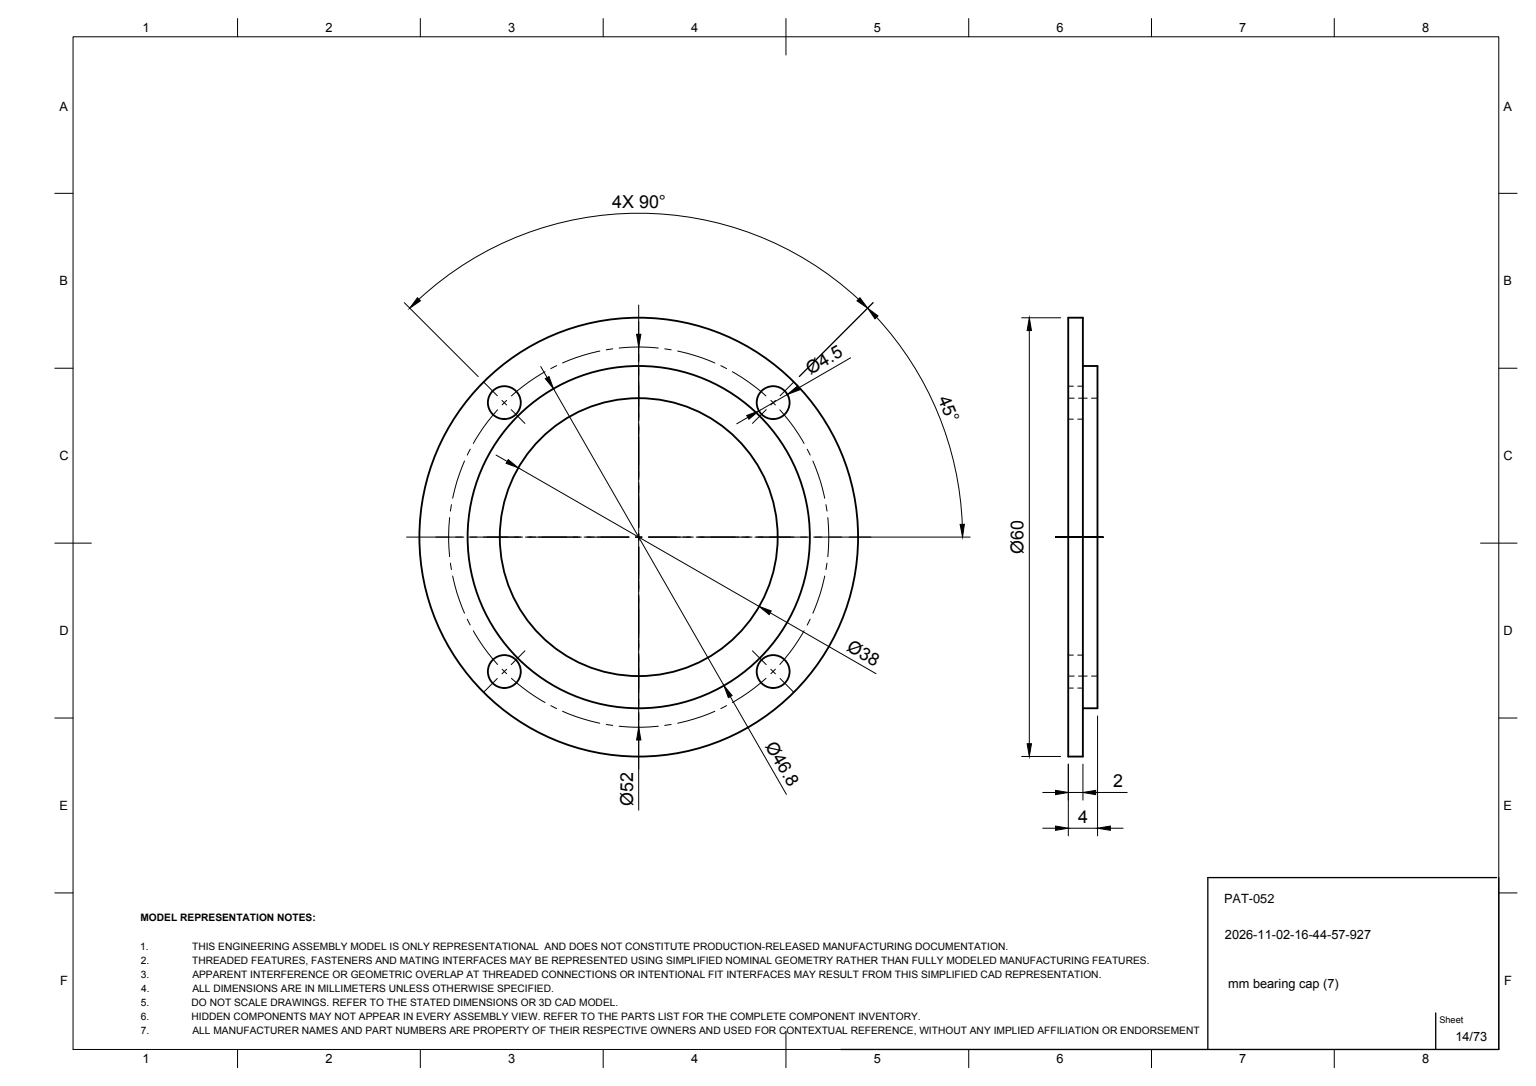
ISO-10303-21;
HEADER;
/* Generated by software containing ST-Developer
 * from STEP Tools, Inc. (www.steptools.com) 
 */

FILE_DESCRIPTION(
/* description */ ('Hand-crank gear train demonstrator'),
/* implementation_level */ '2;1');

FILE_NAME(
/* name */ 'mm bearing cap (7).step',
/* time_stamp */ '2026-10-28T03:22:13-07:00',
/* author */ (''),
/* organization */ (''),
/* preprocessor_version */ 'ST-DEVELOPER v20.2',
/* originating_system */ 'Autodesk Translation Framework v15.17.0.0',
/* authorisation */ '');

FILE_SCHEMA (('AUTOMOTIVE_DESIGN { 1 0 10303 214 3 1 1 }'));
ENDSEC;

DATA;
#10=MECHANICAL_DESIGN_GEOMETRIC_PRESENTATION_REPRESENTATION('',(#1199),#62758);
#1071=SHAPE_REPRESENTATION_RELATIONSHIP('SRR','None',#63043,#1135);
#1135=ADVANCED_BREP_SHAPE_REPRESENTATION('',(#1277),#62697);
#1199=STYLED_ITEM('',(#63462),#1277);
#1277=MANIFOLD_SOLID_BREP('Body1',#16380);
#1476=FACE_BOUND('',#3327,.T.);
#1477=FACE_BOUND('',#3331,.T.);
#1478=FACE_BOUND('',#3332,.T.);
#1479=FACE_BOUND('',#3333,.T.);
#1480=FACE_BOUND('',#3334,.T.);
#1481=FACE_BOUND('',#3335,.T.);
#1482=FACE_BOUND('',#3337,.T.);
#1483=FACE_BOUND('',#3338,.T.);
#1484=FACE_BOUND('',#3339,.T.);
#1485=FACE_BOUND('',#3340,.T.);
#1486=FACE_BOUND('',#3341,.T.);
#1679=PLANE('',#17475);
#1680=PLANE('',#17482);
#1681=PLANE('',#17483);
#2251=FACE_OUTER_BOUND('',#3321,.T.);
#2252=FACE_OUTER_BOUND('',#3322,.T.);
#2253=FACE_OUTER_BOUND('',#3323,.T.);
#2254=FACE_OUTER_BOUND('',#3324,.T.);
#2255=FACE_OUTER_BOUND('',#3325,.T.);
#2256=FACE_OUTER_BOUND('',#3326,.T.);
#2257=FACE_OUTER_BOUND('',#3328,.T.);
#2258=FACE_OUTER_BOUND('',#3329,.T.);
#2259=FACE_OUTER_BOUND('',#3330,.T.);
#2260=FACE_OUTER_BOUND('',#3336,.T.);
#3321=EDGE_LOOP('',(#11417,#11418,#11419,#11420));
#3322=EDGE_LOOP('',(#11421,#11422,#11423,#11424));
#3323=EDGE_LOOP('',(#11425,#11426,#11427,#11428));
#3324=EDGE_LOOP('',(#11429,#11430,#11431,#11432));
#3325=EDGE_LOOP('',(#11433,#11434,#11435,#11436));
#3326=EDGE_LOOP('',(#11437));
#3327=EDGE_LOOP('',(#11438));
#3328=EDGE_LOOP('',(#11439,#11440,#11441,#11442));
#3329=EDGE_LOOP('',(#11443,#11444,#11445,#11446));
#3330=EDGE_LOOP('',(#11447));
#3331=EDGE_LOOP('',(#11448));
#3332=EDGE_LOOP('',(#11449));
#3333=EDGE_LOOP('',(#11450));
#3334=EDGE_LOOP('',(#11451));
#3335=EDGE_LOOP('',(#11452));
#3336=EDGE_LOOP('',(#11453));
#3337=EDGE_LOOP('',(#11454));
#3338=EDGE_LOOP('',(#11455));
#3339=EDGE_LOOP('',(#11456));
#3340=EDGE_LOOP('',(#11457));
#3341=EDGE_LOOP('',(#11458));
#4416=LINE('',#23938,#5548);
#4417=LINE('',#23944,#5549);
#4418=LINE('',#23950,#5550);
#4419=LINE('',#23956,#5551);
#4420=LINE('',#23962,#5552);
#4421=LINE('',#23970,#5553);
#4422=LINE('',#23975,#5554);
#5548=VECTOR('',#19569,0.225000000000001);
#5549=VECTOR('',#19576,0.225000000000001);
#5550=VECTOR('',#19583,0.225000000000001);
#5551=VECTOR('',#19590,0.225000000000001);
#5552=VECTOR('',#19597,2.34);
#5553=VECTOR('',#19608,1.9);
#5554=VECTOR('',#19613,3.);
#6711=CIRCLE('',#17461,0.225000000000001);
#6712=CIRCLE('',#17462,0.225000000000001);
#6713=CIRCLE('',#17464,0.225000000000001);
#6714=CIRCLE('',#17465,0.225000000000001);
#6715=CIRCLE('',#17467,0.225000000000001);
#6716=CIRCLE('',#17468,0.225000000000001);
#6717=CIRCLE('',#17470,0.225000000000001);
#6718=CIRCLE('',#17471,0.225000000000001);
#6719=CIRCLE('',#17473,2.34);
#6720=CIRCLE('',#17474,2.34);
#6721=CIRCLE('',#17476,1.9);
#6722=CIRCLE('',#17478,1.9);
#6723=CIRCLE('',#17480,3.);
#6724=CIRCLE('',#17481,3.);
#7405=VERTEX_POINT('',#23935);
#7406=VERTEX_POINT('',#23937);
#7407=VERTEX_POINT('',#23941);
#7408=VERTEX_POINT('',#23943);
#7409=VERTEX_POINT('',#23947);
#7410=VERTEX_POINT('',#23949);
#7411=VERTEX_POINT('',#23953);
#7412=VERTEX_POINT('',#23955);
#7413=VERTEX_POINT('',#23959);
#7414=VERTEX_POINT('',#23961);
#7415=VERTEX_POINT('',#23965);
#7416=VERTEX_POINT('',#23968);
#7417=VERTEX_POINT('',#23972);
#7418=VERTEX_POINT('',#23974);
#8960=EDGE_CURVE('',#7405,#7405,#6711,.T.);
#8961=EDGE_CURVE('',#7405,#7406,#4416,.T.);
#8962=EDGE_CURVE('',#7406,#7406,#6712,.T.);
#8963=EDGE_CURVE('',#7407,#7407,#6713,.T.);
#8964=EDGE_CURVE('',#7407,#7408,#4417,.T.);
#8965=EDGE_CURVE('',#7408,#7408,#6714,.T.);
#8966=EDGE_CURVE('',#7409,#7409,#6715,.T.);
#8967=EDGE_CURVE('',#7409,#7410,#4418,.T.);
#8968=EDGE_CURVE('',#7410,#7410,#6716,.T.);
#8969=EDGE_CURVE('',#7411,#7411,#6717,.T.);
#8970=EDGE_CURVE('',#7411,#7412,#4419,.T.);
#8971=EDGE_CURVE('',#7412,#7412,#6718,.T.);
#8972=EDGE_CURVE('',#7413,#7413,#6719,.T.);
#8973=EDGE_CURVE('',#7413,#7414,#4420,.T.);
#8974=EDGE_CURVE('',#7414,#7414,#6720,.T.);
#8975=EDGE_CURVE('',#7415,#7415,#6721,.T.);
#8976=EDGE_CURVE('',#7416,#7416,#6722,.T.);
#8977=EDGE_CURVE('',#7416,#7415,#4421,.T.);
#8978=EDGE_CURVE('',#7417,#7417,#6723,.T.);
#8979=EDGE_CURVE('',#7417,#7418,#4422,.T.);
#8980=EDGE_CURVE('',#7418,#7418,#6724,.T.);
#11417=ORIENTED_EDGE('',*,*,#8960,.F.);
#11418=ORIENTED_EDGE('',*,*,#8961,.T.);
#11419=ORIENTED_EDGE('',*,*,#8962,.F.);
#11420=ORIENTED_EDGE('',*,*,#8961,.F.);
#11421=ORIENTED_EDGE('',*,*,#8963,.F.);
#11422=ORIENTED_EDGE('',*,*,#8964,.T.);
#11423=ORIENTED_EDGE('',*,*,#8965,.F.);
#11424=ORIENTED_EDGE('',*,*,#8964,.F.);
#11425=ORIENTED_EDGE('',*,*,#8966,.F.);
#11426=ORIENTED_EDGE('',*,*,#8967,.T.);
#11427=ORIENTED_EDGE('',*,*,#8968,.F.);
#11428=ORIENTED_EDGE('',*,*,#8967,.F.);
#11429=ORIENTED_EDGE('',*,*,#8969,.F.);
#11430=ORIENTED_EDGE('',*,*,#8970,.T.);
#11431=ORIENTED_EDGE('',*,*,#8971,.F.);
#11432=ORIENTED_EDGE('',*,*,#8970,.F.);
#11433=ORIENTED_EDGE('',*,*,#8972,.F.);
#11434=ORIENTED_EDGE('',*,*,#8973,.T.);
#11435=ORIENTED_EDGE('',*,*,#8974,.T.);
#11436=ORIENTED_EDGE('',*,*,#8973,.F.);
#11437=ORIENTED_EDGE('',*,*,#8974,.F.);
#11438=ORIENTED_EDGE('',*,*,#8975,.F.);
#11439=ORIENTED_EDGE('',*,*,#8976,.F.);
#11440=ORIENTED_EDGE('',*,*,#8977,.T.);
#11441=ORIENTED_EDGE('',*,*,#8975,.T.);
#11442=ORIENTED_EDGE('',*,*,#8977,.F.);
#11443=ORIENTED_EDGE('',*,*,#8978,.F.);
#11444=ORIENTED_EDGE('',*,*,#8979,.T.);
#11445=ORIENTED_EDGE('',*,*,#8980,.T.);
#11446=ORIENTED_EDGE('',*,*,#8979,.F.);
#11447=ORIENTED_EDGE('',*,*,#8978,.T.);
#11448=ORIENTED_EDGE('',*,*,#8976,.T.);
#11449=ORIENTED_EDGE('',*,*,#8971,.T.);
#11450=ORIENTED_EDGE('',*,*,#8968,.T.);
#11451=ORIENTED_EDGE('',*,*,#8965,.T.);
#11452=ORIENTED_EDGE('',*,*,#8962,.T.);
#11453=ORIENTED_EDGE('',*,*,#8980,.F.);
#11454=ORIENTED_EDGE('',*,*,#8972,.T.);
#11455=ORIENTED_EDGE('',*,*,#8969,.T.);
#11456=ORIENTED_EDGE('',*,*,#8966,.T.);
#11457=ORIENTED_EDGE('',*,*,#8963,.T.);
#11458=ORIENTED_EDGE('',*,*,#8960,.T.);
#15246=CYLINDRICAL_SURFACE('',#17460,0.225000000000001);
#15247=CYLINDRICAL_SURFACE('',#17463,0.225000000000001);
#15248=CYLINDRICAL_SURFACE('',#17466,0.225000000000001);
#15249=CYLINDRICAL_SURFACE('',#17469,0.225000000000001);
#15250=CYLINDRICAL_SURFACE('',#17472,2.34);
#15251=CYLINDRICAL_SURFACE('',#17477,1.9);
#15252=CYLINDRICAL_SURFACE('',#17479,3.);
#15561=ADVANCED_FACE('',(#2251),#15246,.F.);
#15562=ADVANCED_FACE('',(#2252),#15247,.F.);
#15563=ADVANCED_FACE('',(#2253),#15248,.F.);
#15564=ADVANCED_FACE('',(#2254),#15249,.F.);
#15565=ADVANCED_FACE('',(#2255),#15250,.T.);
#15566=ADVANCED_FACE('',(#2256,#1476),#1679,.F.);
#15567=ADVANCED_FACE('',(#2257),#15251,.F.);
#15568=ADVANCED_FACE('',(#2258),#15252,.T.);
#15569=ADVANCED_FACE('',(#2259,#1477,#1478,#1479,#1480,#1481),#1680,.T.);
#15570=ADVANCED_FACE('',(#2260,#1482,#1483,#1484,#1485,#1486),#1681,.F.);
#16380=CLOSED_SHELL('',(#15561,#15562,#15563,#15564,#15565,#15566,#15567,
#15568,#15569,#15570));
#17459=AXIS2_PLACEMENT_3D('',#23933,#19563,#19564);
#17460=AXIS2_PLACEMENT_3D('',#23934,#19565,#19566);
#17461=AXIS2_PLACEMENT_3D('',#23936,#19567,#19568);
#17462=AXIS2_PLACEMENT_3D('',#23939,#19570,#19571);
#17463=AXIS2_PLACEMENT_3D('',#23940,#19572,#19573);
#17464=AXIS2_PLACEMENT_3D('',#23942,#19574,#19575);
#17465=AXIS2_PLACEMENT_3D('',#23945,#19577,#19578);
#17466=AXIS2_PLACEMENT_3D('',#23946,#19579,#19580);
#17467=AXIS2_PLACEMENT_3D('',#23948,#19581,#19582);
#17468=AXIS2_PLACEMENT_3D('',#23951,#19584,#19585);
#17469=AXIS2_PLACEMENT_3D('',#23952,#19586,#19587);
#17470=AXIS2_PLACEMENT_3D('',#23954,#19588,#19589);
#17471=AXIS2_PLACEMENT_3D('',#23957,#19591,#19592);
#17472=AXIS2_PLACEMENT_3D('',#23958,#19593,#19594);
#17473=AXIS2_PLACEMENT_3D('',#23960,#19595,#19596);
#17474=AXIS2_PLACEMENT_3D('',#23963,#19598,#19599);
#17475=AXIS2_PLACEMENT_3D('',#23964,#19600,#19601);
#17476=AXIS2_PLACEMENT_3D('',#23966,#19602,#19603);
#17477=AXIS2_PLACEMENT_3D('',#23967,#19604,#19605);
#17478=AXIS2_PLACEMENT_3D('',#23969,#19606,#19607);
#17479=AXIS2_PLACEMENT_3D('',#23971,#19609,#19610);
#17480=AXIS2_PLACEMENT_3D('',#23973,#19611,#19612);
#17481=AXIS2_PLACEMENT_3D('',#23976,#19614,#19615);
#17482=AXIS2_PLACEMENT_3D('',#23977,#19616,#19617);
#17483=AXIS2_PLACEMENT_3D('',#23978,#19618,#19619);
#19563=DIRECTION('axis',(0.,0.,1.));
#19564=DIRECTION('refdir',(1.,0.,0.));
#19565=DIRECTION('center_axis',(0.,1.,0.));
#19566=DIRECTION('ref_axis',(1.,0.,0.));
#19567=DIRECTION('center_axis',(0.,1.,0.));
#19568=DIRECTION('ref_axis',(1.,0.,0.));
#19569=DIRECTION('',(0.,1.,0.));
#19570=DIRECTION('center_axis',(0.,-1.,0.));
#19571=DIRECTION('ref_axis',(1.,0.,0.));
#19572=DIRECTION('center_axis',(0.,1.,0.));
#19573=DIRECTION('ref_axis',(1.,0.,0.));
#19574=DIRECTION('center_axis',(0.,1.,0.));
#19575=DIRECTION('ref_axis',(1.,0.,0.));
#19576=DIRECTION('',(0.,1.,0.));
#19577=DIRECTION('center_axis',(0.,-1.,0.));
#19578=DIRECTION('ref_axis',(1.,0.,0.));
#19579=DIRECTION('center_axis',(0.,1.,0.));
#19580=DIRECTION('ref_axis',(1.,0.,0.));
#19581=DIRECTION('center_axis',(0.,1.,0.));
#19582=DIRECTION('ref_axis',(1.,0.,0.));
#19583=DIRECTION('',(0.,1.,0.));
#19584=DIRECTION('center_axis',(0.,-1.,0.));
#19585=DIRECTION('ref_axis',(1.,0.,0.));
#19586=DIRECTION('center_axis',(0.,1.,0.));
#19587=DIRECTION('ref_axis',(1.,0.,0.));
#19588=DIRECTION('center_axis',(0.,1.,0.));
#19589=DIRECTION('ref_axis',(1.,0.,0.));
#19590=DIRECTION('',(0.,1.,0.));
#19591=DIRECTION('center_axis',(0.,-1.,0.));
#19592=DIRECTION('ref_axis',(1.,0.,0.));
#19593=DIRECTION('center_axis',(0.,1.,0.));
#19594=DIRECTION('ref_axis',(1.,0.,0.));
#19595=DIRECTION('center_axis',(0.,1.,0.));
#19596=DIRECTION('ref_axis',(1.,0.,0.));
#19597=DIRECTION('',(0.,-1.,0.));
#19598=DIRECTION('center_axis',(0.,1.,0.));
#19599=DIRECTION('ref_axis',(1.,0.,0.));
#19600=DIRECTION('center_axis',(0.,1.,0.));
#19601=DIRECTION('ref_axis',(1.,0.,0.));
#19602=DIRECTION('center_axis',(0.,-1.,0.));
#19603=DIRECTION('ref_axis',(1.,0.,0.));
#19604=DIRECTION('center_axis',(0.,1.,0.));
#19605=DIRECTION('ref_axis',(1.,0.,0.));
#19606=DIRECTION('center_axis',(0.,-1.,0.));
#19607=DIRECTION('ref_axis',(1.,0.,0.));
#19608=DIRECTION('',(0.,-1.,0.));
#19609=DIRECTION('center_axis',(0.,1.,0.));
#19610=DIRECTION('ref_axis',(1.,0.,0.));
#19611=DIRECTION('center_axis',(0.,1.,0.));
#19612=DIRECTION('ref_axis',(1.,0.,0.));
#19613=DIRECTION('',(0.,-1.,0.));
#19614=DIRECTION('center_axis',(0.,1.,0.));
#19615=DIRECTION('ref_axis',(1.,0.,0.));
#19616=DIRECTION('center_axis',(0.,1.,0.));
#19617=DIRECTION('ref_axis',(1.,0.,0.));
#19618=DIRECTION('center_axis',(0.,1.,0.));
#19619=DIRECTION('ref_axis',(1.,0.,0.));
#23933=CARTESIAN_POINT('',(0.,0.,0.));
#23934=CARTESIAN_POINT('Origin',(16.161522368915,-0.7,7.16152236891498));
#23935=CARTESIAN_POINT('',(15.936522368915,-0.6,7.16152236891498));
#23936=CARTESIAN_POINT('Origin',(16.161522368915,-0.6,7.16152236891498));
#23937=CARTESIAN_POINT('',(15.936522368915,-0.4,7.16152236891498));
#23938=CARTESIAN_POINT('',(15.936522368915,-0.7,7.16152236891498));
#23939=CARTESIAN_POINT('Origin',(16.161522368915,-0.4,7.16152236891498));
#23940=CARTESIAN_POINT('Origin',(16.161522368915,-0.7,10.838477631085));
#23941=CARTESIAN_POINT('',(15.936522368915,-0.6,10.838477631085));
#23942=CARTESIAN_POINT('Origin',(16.161522368915,-0.6,10.838477631085));
#23943=CARTESIAN_POINT('',(15.936522368915,-0.4,10.838477631085));
#23944=CARTESIAN_POINT('',(15.936522368915,-0.7,10.838477631085));
#23945=CARTESIAN_POINT('Origin',(16.161522368915,-0.4,10.838477631085));
#23946=CARTESIAN_POINT('Origin',(19.838477631085,-0.7,10.838477631085));
#23947=CARTESIAN_POINT('',(19.613477631085,-0.6,10.838477631085));
#23948=CARTESIAN_POINT('Origin',(19.838477631085,-0.6,10.838477631085));
#23949=CARTESIAN_POINT('',(19.613477631085,-0.4,10.838477631085));
#23950=CARTESIAN_POINT('',(19.613477631085,-0.7,10.838477631085));
#23951=CARTESIAN_POINT('Origin',(19.838477631085,-0.4,10.838477631085));
#23952=CARTESIAN_POINT('Origin',(19.838477631085,-0.7,7.16152236891498));
#23953=CARTESIAN_POINT('',(19.613477631085,-0.6,7.16152236891498));
#23954=CARTESIAN_POINT('Origin',(19.838477631085,-0.6,7.16152236891498));
#23955=CARTESIAN_POINT('',(19.613477631085,-0.4,7.16152236891498));
#23956=CARTESIAN_POINT('',(19.613477631085,-0.7,7.16152236891498));
#23957=CARTESIAN_POINT('Origin',(19.838477631085,-0.4,7.16152236891498));
#23958=CARTESIAN_POINT('Origin',(18.,-0.8,9.));
#23959=CARTESIAN_POINT('',(15.66,-0.6,9.));
#23960=CARTESIAN_POINT('Origin',(18.,-0.6,9.));
#23961=CARTESIAN_POINT('',(15.66,-0.8,9.));
#23962=CARTESIAN_POINT('',(15.66,-0.8,9.));
#23963=CARTESIAN_POINT('Origin',(18.,-0.8,9.));
#23964=CARTESIAN_POINT('Origin',(18.,-0.8,9.));
#23965=CARTESIAN_POINT('',(16.1,-0.8,9.));
#23966=CARTESIAN_POINT('Origin',(18.,-0.8,9.));
#23967=CARTESIAN_POINT('Origin',(18.,-0.6,9.));
#23968=CARTESIAN_POINT('',(16.1,-0.4,9.));
#23969=CARTESIAN_POINT('Origin',(18.,-0.4,9.));
#23970=CARTESIAN_POINT('',(16.1,-0.6,9.));
#23971=CARTESIAN_POINT('Origin',(18.,-0.6,9.));
#23972=CARTESIAN_POINT('',(15.,-0.4,9.));
#23973=CARTESIAN_POINT('Origin',(18.,-0.4,9.));
#23974=CARTESIAN_POINT('',(15.,-0.6,9.));
#23975=CARTESIAN_POINT('',(15.,-0.6,9.));
#23976=CARTESIAN_POINT('Origin',(18.,-0.6,9.));
#23977=CARTESIAN_POINT('Origin',(18.,-0.4,9.));
#23978=CARTESIAN_POINT('Origin',(18.,-0.6,9.));
#62623=UNCERTAINTY_MEASURE_WITH_UNIT(LENGTH_MEASURE(0.001),#62759,
'DISTANCE_ACCURACY_VALUE',
'Maximum model space distance between geometric entities at asserted c
onnectivities');
#62684=UNCERTAINTY_MEASURE_WITH_UNIT(LENGTH_MEASURE(0.001),#62759,
'DISTANCE_ACCURACY_VALUE',
'Maximum model space distance between geometric entities at asserted c
onnectivities');
#62697=(
GEOMETRIC_REPRESENTATION_CONTEXT(3)
GLOBAL_UNCERTAINTY_ASSIGNED_CONTEXT((#62623))
GLOBAL_UNIT_ASSIGNED_CONTEXT((#62759,#62761,#62762))
REPRESENTATION_CONTEXT('','3D')
);
#62758=(
GEOMETRIC_REPRESENTATION_CONTEXT(3)
GLOBAL_UNCERTAINTY_ASSIGNED_CONTEXT((#62684))
GLOBAL_UNIT_ASSIGNED_CONTEXT((#62759,#62761,#62762))
REPRESENTATION_CONTEXT('','3D')
);
#62759=(
LENGTH_UNIT()
NAMED_UNIT(*)
SI_UNIT(.CENTI.,.METRE.)
);
#62761=(
NAMED_UNIT(*)
PLANE_ANGLE_UNIT()
SI_UNIT($,.RADIAN.)
);
#62762=(
NAMED_UNIT(*)
SI_UNIT($,.STERADIAN.)
SOLID_ANGLE_UNIT()
);
#62775=SHAPE_DEFINITION_REPRESENTATION(#62848,#63043);
#62848=PRODUCT_DEFINITION_SHAPE('',$,#63117);
#63043=SHAPE_REPRESENTATION('',(#17459),#62697);
#63104=PRODUCT_DEFINITION_CONTEXT('part definition',#63325,'design');
#63117=PRODUCT_DEFINITION('mm bearing cap (7)','mm bearing cap (7)',#63190,
#63104);
#63190=PRODUCT_DEFINITION_FORMATION('',$,#63339);
#63325=APPLICATION_CONTEXT(
'Core Data for Automotive Mechanical Design Process');
#63326=PRODUCT_CONTEXT('part definition',#63325,'mechanical');
#63339=PRODUCT('mm bearing cap (7)','mm bearing cap (7)','mm bearing cap (7)',
(#63326));
#63456=COLOUR_RGB('Grey',0.48,0.52,0.57);
#63457=FILL_AREA_STYLE_COLOUR('',#63456);
#63458=FILL_AREA_STYLE('',(#63457));
#63459=SURFACE_STYLE_FILL_AREA(#63458);
#63460=SURFACE_SIDE_STYLE('',(#63459));
#63461=SURFACE_STYLE_USAGE(.BOTH.,#63460);
#63462=PRESENTATION_STYLE_ASSIGNMENT((#63461));
ENDSEC;
END-ISO-10303-21;
